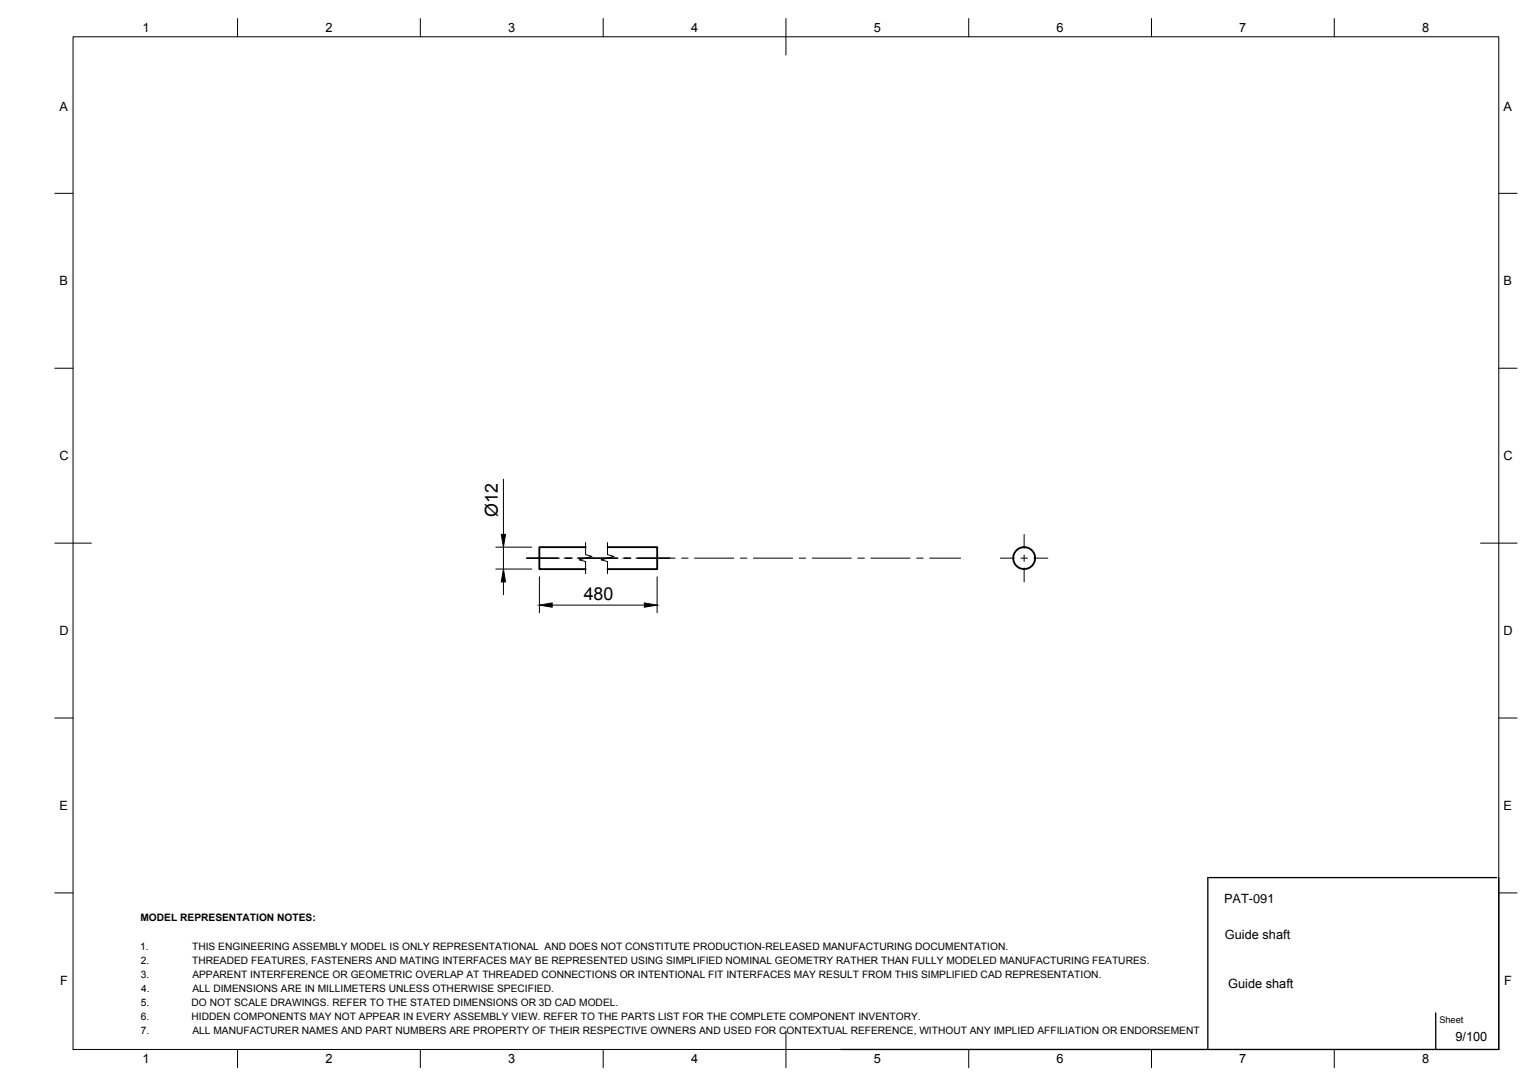
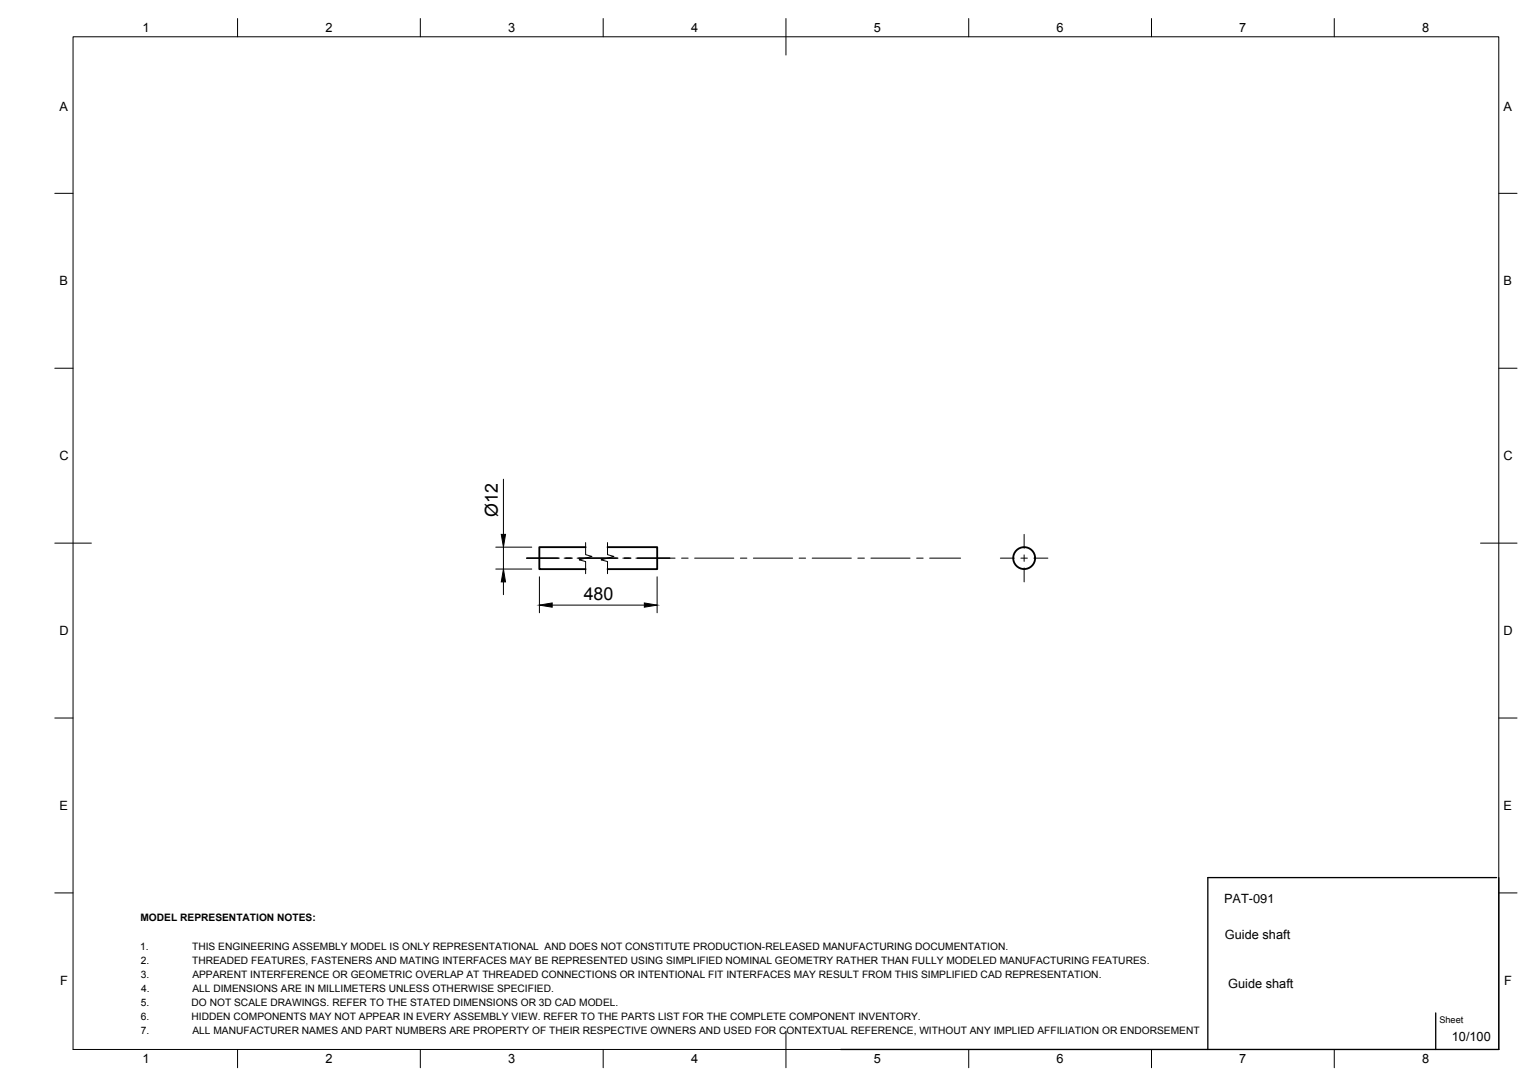
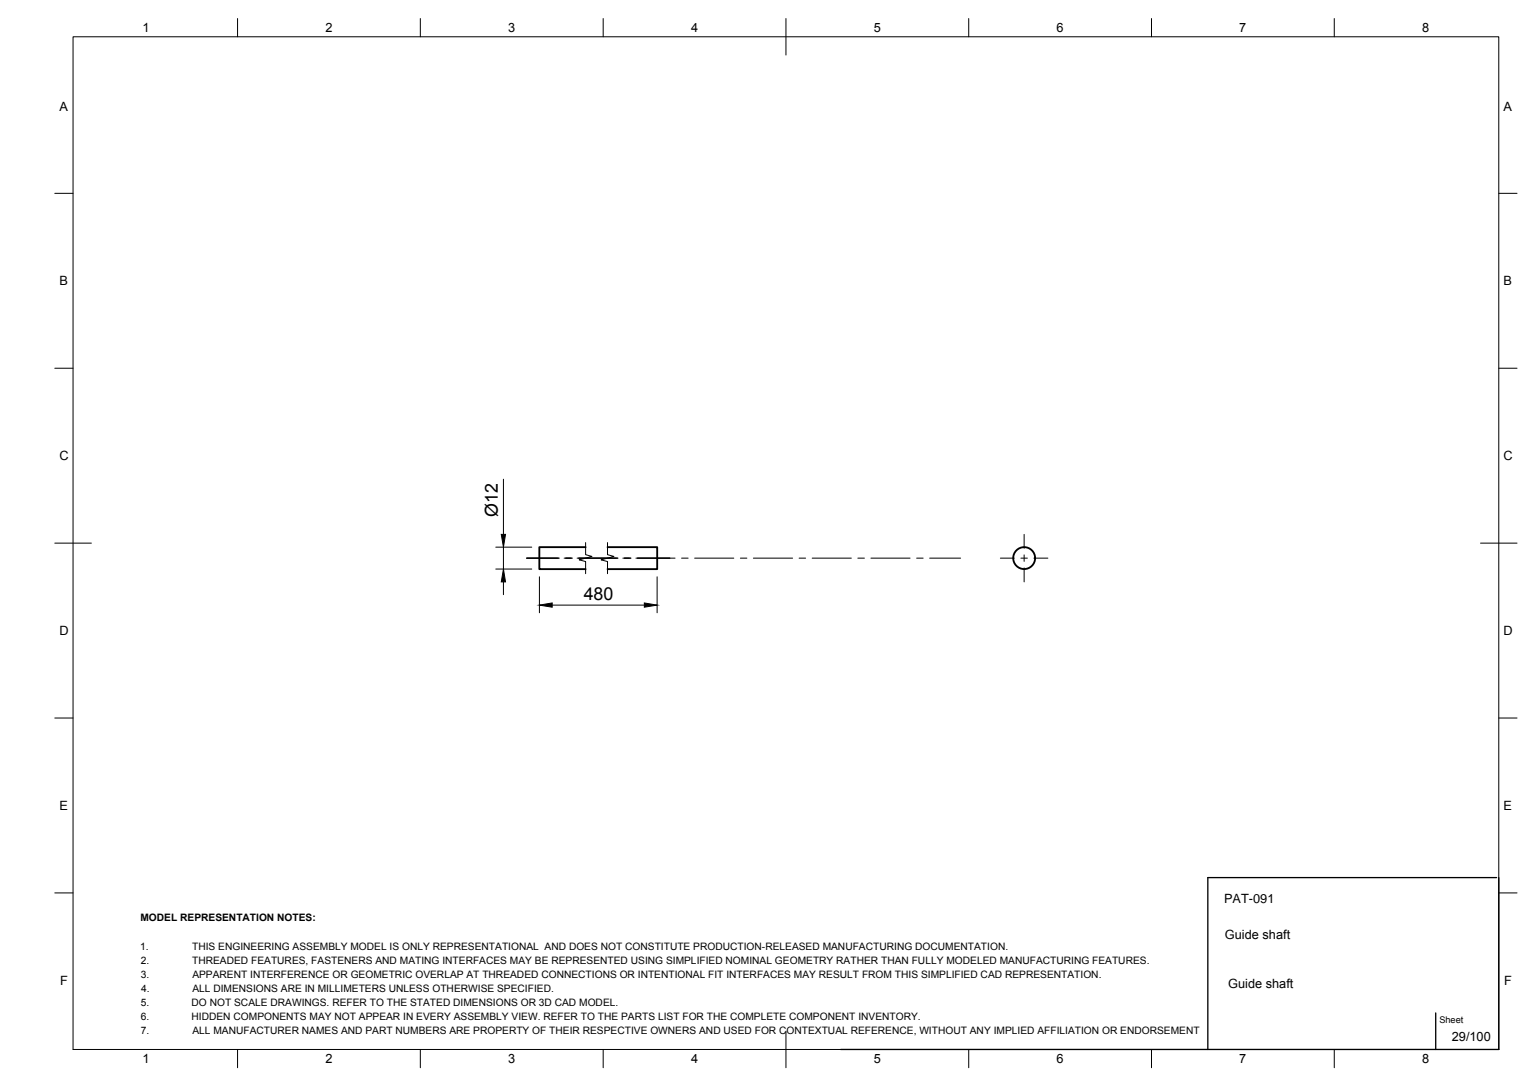
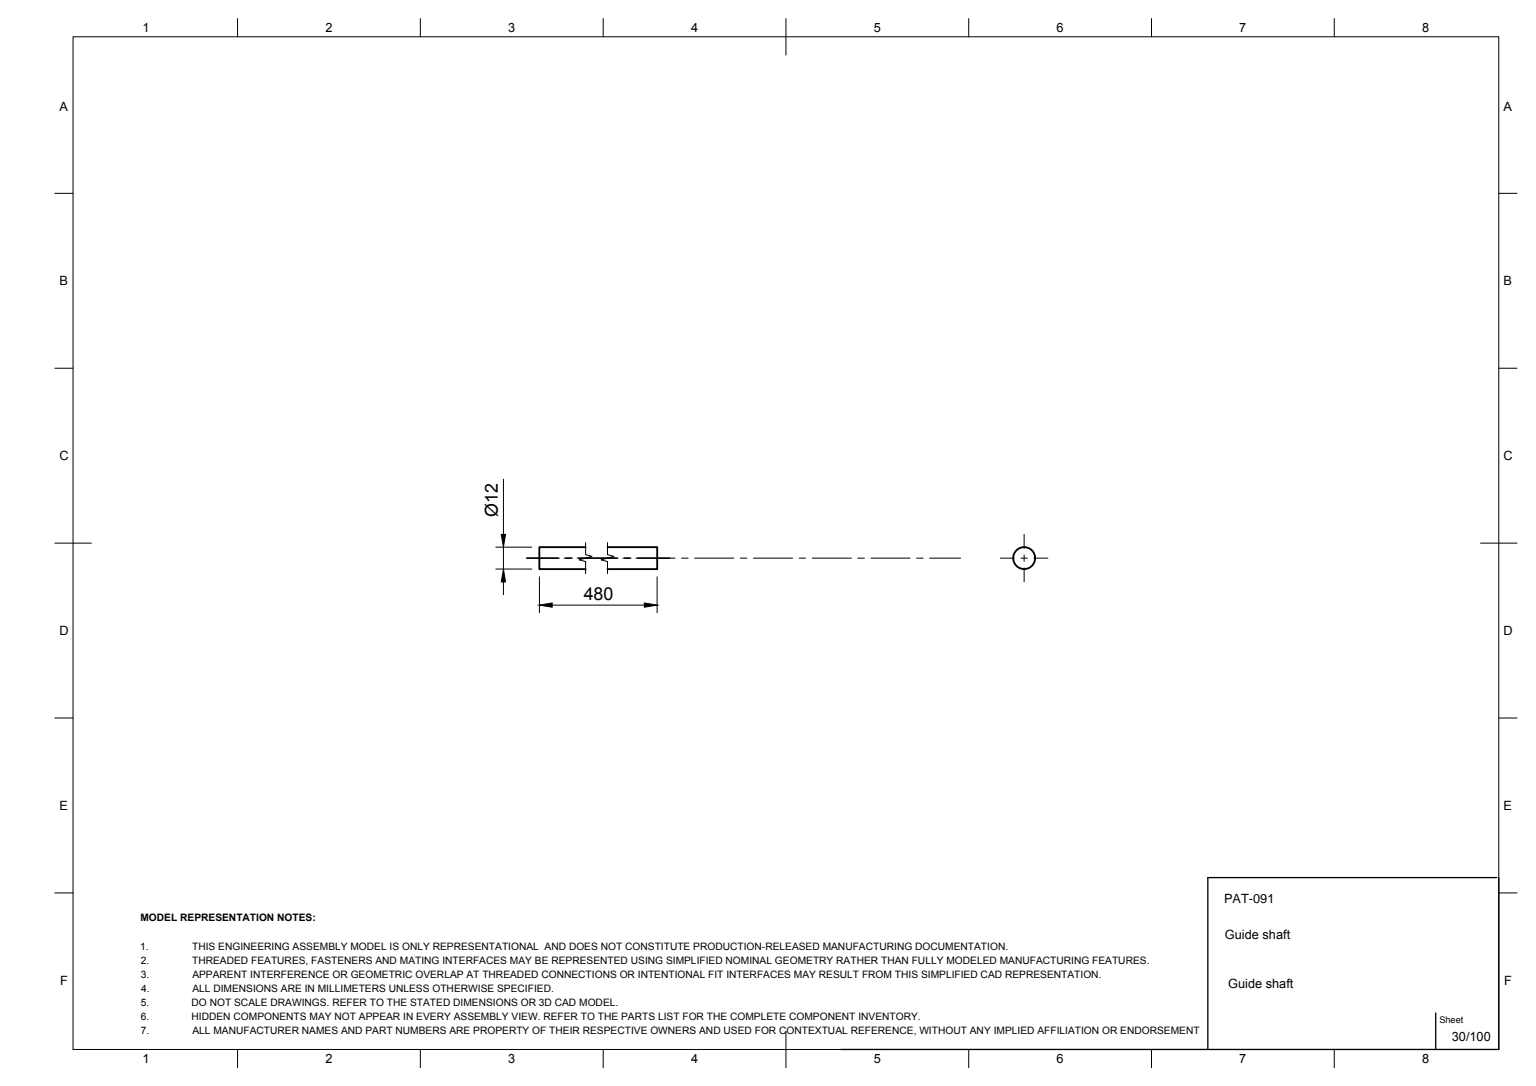
ISO-10303-21;
HEADER;
/* Generated by software containing ST-Developer
 * from STEP Tools, Inc. (www.steptools.com) 
 */

FILE_DESCRIPTION(
/* description */ ('PAT-091'),
/* implementation_level */ '2;1');

FILE_NAME(
/* name */ 'Guide shaft.step',
/* time_stamp */ '2026-10-27T15:34:44-07:00',
/* author */ (''),
/* organization */ (''),
/* preprocessor_version */ 'ST-DEVELOPER v20.2',
/* originating_system */ 'Autodesk Translation Framework v15.17.0.0',
/* authorisation */ '');

FILE_SCHEMA (('AUTOMOTIVE_DESIGN { 1 0 10303 214 3 1 1 }'));
ENDSEC;

DATA;
#10=MECHANICAL_DESIGN_GEOMETRIC_PRESENTATION_REPRESENTATION('',(#980),#25100);
#760=SHAPE_REPRESENTATION_RELATIONSHIP('SRR','None',#25521,#870);
#870=ADVANCED_BREP_SHAPE_REPRESENTATION('',(#1104),#24991);
#980=STYLED_ITEM('',(#26191),#1104);
#1104=MANIFOLD_SOLID_BREP('Body1',#13257);
#1690=PLANE('',#14827);
#1691=PLANE('',#14828);
#2172=FACE_OUTER_BOUND('',#3096,.T.);
#2173=FACE_OUTER_BOUND('',#3097,.T.);
#2174=FACE_OUTER_BOUND('',#3098,.T.);
#3096=EDGE_LOOP('',(#9494,#9495,#9496,#9497));
#3097=EDGE_LOOP('',(#9498));
#3098=EDGE_LOOP('',(#9499));
#4267=LINE('',#21534,#5007);
#5007=VECTOR('',#17093,0.6);
#5722=CIRCLE('',#14825,0.6);
#5723=CIRCLE('',#14826,0.6);
#6557=VERTEX_POINT('',#21531);
#6558=VERTEX_POINT('',#21533);
#7682=EDGE_CURVE('',#6557,#6557,#5722,.T.);
#7683=EDGE_CURVE('',#6557,#6558,#4267,.T.);
#7684=EDGE_CURVE('',#6558,#6558,#5723,.T.);
#9494=ORIENTED_EDGE('',*,*,#7682,.F.);
#9495=ORIENTED_EDGE('',*,*,#7683,.T.);
#9496=ORIENTED_EDGE('',*,*,#7684,.T.);
#9497=ORIENTED_EDGE('',*,*,#7683,.F.);
#9498=ORIENTED_EDGE('',*,*,#7682,.T.);
#9499=ORIENTED_EDGE('',*,*,#7684,.F.);
#12133=CYLINDRICAL_SURFACE('',#14824,0.6);
#12539=ADVANCED_FACE('',(#2172),#12133,.T.);
#12540=ADVANCED_FACE('',(#2173),#1690,.T.);
#12541=ADVANCED_FACE('',(#2174),#1691,.F.);
#13257=CLOSED_SHELL('',(#12539,#12540,#12541));
#14823=AXIS2_PLACEMENT_3D('',#21529,#17087,#17088);
#14824=AXIS2_PLACEMENT_3D('',#21530,#17089,#17090);
#14825=AXIS2_PLACEMENT_3D('',#21532,#17091,#17092);
#14826=AXIS2_PLACEMENT_3D('',#21535,#17094,#17095);
#14827=AXIS2_PLACEMENT_3D('',#21536,#17096,#17097);
#14828=AXIS2_PLACEMENT_3D('',#21537,#17098,#17099);
#17087=DIRECTION('axis',(0.,0.,1.));
#17088=DIRECTION('refdir',(1.,0.,0.));
#17089=DIRECTION('center_axis',(1.,0.,0.));
#17090=DIRECTION('ref_axis',(0.,0.,-1.));
#17091=DIRECTION('center_axis',(1.,0.,0.));
#17092=DIRECTION('ref_axis',(0.,0.,-1.));
#17093=DIRECTION('',(-1.,0.,0.));
#17094=DIRECTION('center_axis',(1.,0.,0.));
#17095=DIRECTION('ref_axis',(0.,0.,-1.));
#17096=DIRECTION('center_axis',(1.,0.,0.));
#17097=DIRECTION('ref_axis',(0.,0.,-1.));
#17098=DIRECTION('center_axis',(1.,0.,0.));
#17099=DIRECTION('ref_axis',(0.,0.,-1.));
#21529=CARTESIAN_POINT('',(0.,0.,0.));
#21530=CARTESIAN_POINT('Origin',(-1.,-3.,6.));
#21531=CARTESIAN_POINT('',(47.,-3.,6.6));
#21532=CARTESIAN_POINT('Origin',(47.,-3.,6.));
#21533=CARTESIAN_POINT('',(-1.,-3.,6.6));
#21534=CARTESIAN_POINT('',(-1.,-3.,6.6));
#21535=CARTESIAN_POINT('Origin',(-1.,-3.,6.));
#21536=CARTESIAN_POINT('Origin',(47.,-3.,6.));
#21537=CARTESIAN_POINT('Origin',(-1.,-3.,6.));
#24870=UNCERTAINTY_MEASURE_WITH_UNIT(LENGTH_MEASURE(0.001),#25101,
'DISTANCE_ACCURACY_VALUE',
'Maximum model space distance between geometric entities at asserted c
onnectivities');
#24979=UNCERTAINTY_MEASURE_WITH_UNIT(LENGTH_MEASURE(0.001),#25101,
'DISTANCE_ACCURACY_VALUE',
'Maximum model space distance between geometric entities at asserted c
onnectivities');
#24991=(
GEOMETRIC_REPRESENTATION_CONTEXT(3)
GLOBAL_UNCERTAINTY_ASSIGNED_CONTEXT((#24870))
GLOBAL_UNIT_ASSIGNED_CONTEXT((#25101,#25103,#25104))
REPRESENTATION_CONTEXT('','3D')
);
#25100=(
GEOMETRIC_REPRESENTATION_CONTEXT(3)
GLOBAL_UNCERTAINTY_ASSIGNED_CONTEXT((#24979))
GLOBAL_UNIT_ASSIGNED_CONTEXT((#25101,#25103,#25104))
REPRESENTATION_CONTEXT('','3D')
);
#25101=(
LENGTH_UNIT()
NAMED_UNIT(*)
SI_UNIT(.CENTI.,.METRE.)
);
#25103=(
NAMED_UNIT(*)
PLANE_ANGLE_UNIT()
SI_UNIT($,.RADIAN.)
);
#25104=(
NAMED_UNIT(*)
SI_UNIT($,.STERADIAN.)
SOLID_ANGLE_UNIT()
);
#25116=SHAPE_DEFINITION_REPRESENTATION(#25236,#25521);
#25236=PRODUCT_DEFINITION_SHAPE('',$,#25642);
#25521=SHAPE_REPRESENTATION('',(#14823),#24991);
#25630=PRODUCT_DEFINITION_CONTEXT('part definition',#25992,'design');
#25642=PRODUCT_DEFINITION('Guide shaft','Guide shaft',#25762,#25630);
#25762=PRODUCT_DEFINITION_FORMATION('',$,#26005);
#25992=APPLICATION_CONTEXT(
'Core Data for Automotive Mechanical Design Process');
#25993=PRODUCT_CONTEXT('part definition',#25992,'mechanical');
#26005=PRODUCT('Guide shaft','Guide shaft','Guide shaft',(#25993));
#26185=COLOUR_RGB('Grey',0.48,0.52,0.57);
#26186=FILL_AREA_STYLE_COLOUR('',#26185);
#26187=FILL_AREA_STYLE('',(#26186));
#26188=SURFACE_STYLE_FILL_AREA(#26187);
#26189=SURFACE_SIDE_STYLE('',(#26188));
#26190=SURFACE_STYLE_USAGE(.BOTH.,#26189);
#26191=PRESENTATION_STYLE_ASSIGNMENT((#26190));
ENDSEC;
END-ISO-10303-21;
